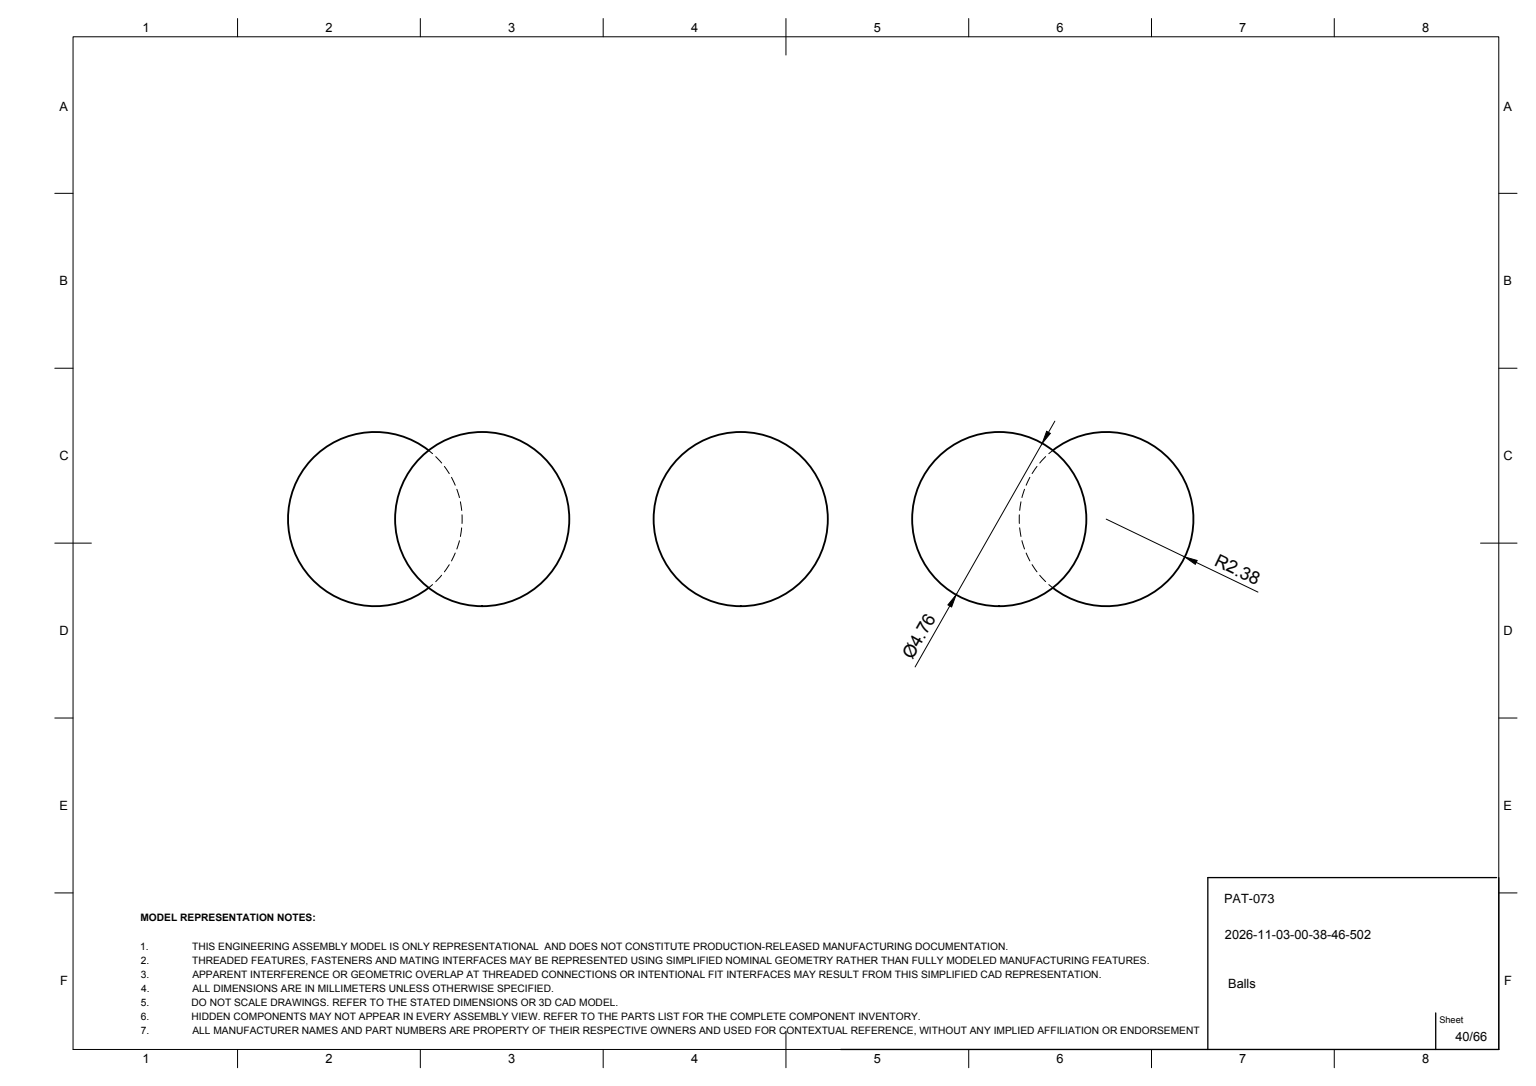
ISO-10303-21;
HEADER;
/* Generated by software containing ST-Developer
 * from STEP Tools, Inc. (www.steptools.com) 
 */

FILE_DESCRIPTION(
/* description */ ('Manual piston pump'),
/* implementation_level */ '2;1');

FILE_NAME(
/* name */ 'Balls.step',
/* time_stamp */ '2026-11-02T16:54:23-08:00',
/* author */ (''),
/* organization */ (''),
/* preprocessor_version */ 'ST-DEVELOPER v20.2',
/* originating_system */ 'Autodesk Translation Framework v15.17.0.0',
/* authorisation */ '');

FILE_SCHEMA (('AUTOMOTIVE_DESIGN { 1 0 10303 214 3 1 1 }'));
ENDSEC;

DATA;
#10=MECHANICAL_DESIGN_GEOMETRIC_PRESENTATION_REPRESENTATION('',(#713,#714,#715,#716,#717,#718,#719,#720),#19043);
#492=SPHERICAL_SURFACE('',#10746,0.23815);
#493=SPHERICAL_SURFACE('',#10748,0.23815);
#494=SPHERICAL_SURFACE('',#10750,0.23815);
#495=SPHERICAL_SURFACE('',#10752,0.23815);
#496=SPHERICAL_SURFACE('',#10754,0.23815);
#497=SPHERICAL_SURFACE('',#10756,0.23815);
#498=SPHERICAL_SURFACE('',#10758,0.23815);
#499=SPHERICAL_SURFACE('',#10760,0.23815);
#587=SHAPE_REPRESENTATION_RELATIONSHIP('SRR','None',#19334,#650);
#650=ADVANCED_BREP_SHAPE_REPRESENTATION('',(#783,#784,#785,#786,#787,#788,
#789,#790),#19001);
#713=STYLED_ITEM('',(#19664),#783);
#714=STYLED_ITEM('',(#19664),#784);
#715=STYLED_ITEM('',(#19664),#785);
#716=STYLED_ITEM('',(#19664),#786);
#717=STYLED_ITEM('',(#19664),#787);
#718=STYLED_ITEM('',(#19664),#788);
#719=STYLED_ITEM('',(#19664),#789);
#720=STYLED_ITEM('',(#19664),#790);
#783=MANIFOLD_SOLID_BREP('Body1',#9499);
#784=MANIFOLD_SOLID_BREP('Body2',#9500);
#785=MANIFOLD_SOLID_BREP('Body3',#9501);
#786=MANIFOLD_SOLID_BREP('Body4',#9502);
#787=MANIFOLD_SOLID_BREP('Body5',#9503);
#788=MANIFOLD_SOLID_BREP('Body6',#9504);
#789=MANIFOLD_SOLID_BREP('Body7',#9505);
#790=MANIFOLD_SOLID_BREP('Body8',#9506);
#1546=FACE_OUTER_BOUND('',#2244,.T.);
#1547=FACE_OUTER_BOUND('',#2245,.T.);
#1548=FACE_OUTER_BOUND('',#2246,.T.);
#1549=FACE_OUTER_BOUND('',#2247,.T.);
#1550=FACE_OUTER_BOUND('',#2248,.T.);
#1551=FACE_OUTER_BOUND('',#2249,.T.);
#1552=FACE_OUTER_BOUND('',#2250,.T.);
#1553=FACE_OUTER_BOUND('',#2251,.T.);
#2244=EDGE_LOOP('',(#7313,#7314));
#2245=EDGE_LOOP('',(#7315,#7316));
#2246=EDGE_LOOP('',(#7317,#7318));
#2247=EDGE_LOOP('',(#7319,#7320));
#2248=EDGE_LOOP('',(#7321,#7322));
#2249=EDGE_LOOP('',(#7323,#7324));
#2250=EDGE_LOOP('',(#7325,#7326));
#2251=EDGE_LOOP('',(#7327,#7328));
#2883=CIRCLE('',#10747,0.23815);
#2884=CIRCLE('',#10749,0.23815);
#2885=CIRCLE('',#10751,0.23815);
#2886=CIRCLE('',#10753,0.23815);
#2887=CIRCLE('',#10755,0.23815);
#2888=CIRCLE('',#10757,0.23815);
#2889=CIRCLE('',#10759,0.23815);
#2890=CIRCLE('',#10761,0.23815);
#4696=VERTEX_POINT('',#15823);
#4697=VERTEX_POINT('',#15824);
#4698=VERTEX_POINT('',#15827);
#4699=VERTEX_POINT('',#15828);
#4700=VERTEX_POINT('',#15831);
#4701=VERTEX_POINT('',#15832);
#4702=VERTEX_POINT('',#15835);
#4703=VERTEX_POINT('',#15836);
#4704=VERTEX_POINT('',#15839);
#4705=VERTEX_POINT('',#15840);
#4706=VERTEX_POINT('',#15843);
#4707=VERTEX_POINT('',#15844);
#4708=VERTEX_POINT('',#15847);
#4709=VERTEX_POINT('',#15848);
#4710=VERTEX_POINT('',#15851);
#4711=VERTEX_POINT('',#15852);
#5643=EDGE_CURVE('',#4696,#4697,#2883,.T.);
#5644=EDGE_CURVE('',#4698,#4699,#2884,.T.);
#5645=EDGE_CURVE('',#4700,#4701,#2885,.T.);
#5646=EDGE_CURVE('',#4702,#4703,#2886,.T.);
#5647=EDGE_CURVE('',#4704,#4705,#2887,.T.);
#5648=EDGE_CURVE('',#4706,#4707,#2888,.T.);
#5649=EDGE_CURVE('',#4708,#4709,#2889,.T.);
#5650=EDGE_CURVE('',#4710,#4711,#2890,.T.);
#7313=ORIENTED_EDGE('',*,*,#5643,.T.);
#7314=ORIENTED_EDGE('',*,*,#5643,.F.);
#7315=ORIENTED_EDGE('',*,*,#5644,.T.);
#7316=ORIENTED_EDGE('',*,*,#5644,.F.);
#7317=ORIENTED_EDGE('',*,*,#5645,.T.);
#7318=ORIENTED_EDGE('',*,*,#5645,.F.);
#7319=ORIENTED_EDGE('',*,*,#5646,.T.);
#7320=ORIENTED_EDGE('',*,*,#5646,.F.);
#7321=ORIENTED_EDGE('',*,*,#5647,.T.);
#7322=ORIENTED_EDGE('',*,*,#5647,.F.);
#7323=ORIENTED_EDGE('',*,*,#5648,.T.);
#7324=ORIENTED_EDGE('',*,*,#5648,.F.);
#7325=ORIENTED_EDGE('',*,*,#5649,.T.);
#7326=ORIENTED_EDGE('',*,*,#5649,.F.);
#7327=ORIENTED_EDGE('',*,*,#5650,.T.);
#7328=ORIENTED_EDGE('',*,*,#5650,.F.);
#9151=ADVANCED_FACE('',(#1546),#492,.T.);
#9152=ADVANCED_FACE('',(#1547),#493,.T.);
#9153=ADVANCED_FACE('',(#1548),#494,.T.);
#9154=ADVANCED_FACE('',(#1549),#495,.T.);
#9155=ADVANCED_FACE('',(#1550),#496,.T.);
#9156=ADVANCED_FACE('',(#1551),#497,.T.);
#9157=ADVANCED_FACE('',(#1552),#498,.T.);
#9158=ADVANCED_FACE('',(#1553),#499,.T.);
#9499=CLOSED_SHELL('',(#9151));
#9500=CLOSED_SHELL('',(#9152));
#9501=CLOSED_SHELL('',(#9153));
#9502=CLOSED_SHELL('',(#9154));
#9503=CLOSED_SHELL('',(#9155));
#9504=CLOSED_SHELL('',(#9156));
#9505=CLOSED_SHELL('',(#9157));
#9506=CLOSED_SHELL('',(#9158));
#10745=AXIS2_PLACEMENT_3D('',#15821,#12784,#12785);
#10746=AXIS2_PLACEMENT_3D('',#15822,#12786,#12787);
#10747=AXIS2_PLACEMENT_3D('',#15825,#12788,#12789);
#10748=AXIS2_PLACEMENT_3D('',#15826,#12790,#12791);
#10749=AXIS2_PLACEMENT_3D('',#15829,#12792,#12793);
#10750=AXIS2_PLACEMENT_3D('',#15830,#12794,#12795);
#10751=AXIS2_PLACEMENT_3D('',#15833,#12796,#12797);
#10752=AXIS2_PLACEMENT_3D('',#15834,#12798,#12799);
#10753=AXIS2_PLACEMENT_3D('',#15837,#12800,#12801);
#10754=AXIS2_PLACEMENT_3D('',#15838,#12802,#12803);
#10755=AXIS2_PLACEMENT_3D('',#15841,#12804,#12805);
#10756=AXIS2_PLACEMENT_3D('',#15842,#12806,#12807);
#10757=AXIS2_PLACEMENT_3D('',#15845,#12808,#12809);
#10758=AXIS2_PLACEMENT_3D('',#15846,#12810,#12811);
#10759=AXIS2_PLACEMENT_3D('',#15849,#12812,#12813);
#10760=AXIS2_PLACEMENT_3D('',#15850,#12814,#12815);
#10761=AXIS2_PLACEMENT_3D('',#15853,#12816,#12817);
#12784=DIRECTION('axis',(0.,0.,1.));
#12785=DIRECTION('refdir',(1.,0.,0.));
#12786=DIRECTION('center_axis',(0.,0.,1.));
#12787=DIRECTION('ref_axis',(1.,0.,0.));
#12788=DIRECTION('center_axis',(1.22464679914735E-16,-1.,0.));
#12789=DIRECTION('ref_axis',(-1.,-1.22464679914735E-16,0.));
#12790=DIRECTION('center_axis',(0.707106781186548,0.,0.707106781186548));
#12791=DIRECTION('ref_axis',(0.707106781186548,0.,-0.707106781186548));
#12792=DIRECTION('center_axis',(8.65956056235494E-17,-1.,-8.65956056235493E-17));
#12793=DIRECTION('ref_axis',(-0.707106781186547,-1.22464679914735E-16,0.707106781186547));
#12794=DIRECTION('center_axis',(1.,0.,0.));
#12795=DIRECTION('ref_axis',(6.12323399573676E-17,0.,-1.));
#12796=DIRECTION('center_axis',(7.49879891330929E-33,-1.,-1.22464679914735E-16));
#12797=DIRECTION('ref_axis',(-6.12323399573676E-17,-1.22464679914735E-16,
1.));
#12798=DIRECTION('center_axis',(0.707106781186548,0.,-0.707106781186548));
#12799=DIRECTION('ref_axis',(-0.707106781186548,0.,-0.707106781186548));
#12800=DIRECTION('center_axis',(-8.65956056235493E-17,-1.,-8.65956056235494E-17));
#12801=DIRECTION('ref_axis',(0.707106781186547,-1.22464679914735E-16,0.707106781186547));
#12802=DIRECTION('center_axis',(0.,0.,-1.));
#12803=DIRECTION('ref_axis',(-1.,0.,-1.22464679914735E-16));
#12804=DIRECTION('center_axis',(-1.22464679914735E-16,-1.,-1.49975978266186E-32));
#12805=DIRECTION('ref_axis',(1.,-1.22464679914735E-16,1.22464679914735E-16));
#12806=DIRECTION('center_axis',(-0.707106781186547,0.,-0.707106781186548));
#12807=DIRECTION('ref_axis',(-0.707106781186548,0.,0.707106781186547));
#12808=DIRECTION('center_axis',(-8.65956056235493E-17,-1.,8.65956056235493E-17));
#12809=DIRECTION('ref_axis',(0.707106781186548,-1.22464679914735E-16,-0.707106781186547));
#12810=DIRECTION('center_axis',(-1.,0.,0.));
#12811=DIRECTION('ref_axis',(-1.83697019872103E-16,0.,1.));
#12812=DIRECTION('center_axis',(-2.24963967399279E-32,-1.,1.22464679914735E-16));
#12813=DIRECTION('ref_axis',(1.83697019872103E-16,-1.22464679914735E-16,
-1.));
#12814=DIRECTION('center_axis',(-0.707106781186548,0.,0.707106781186548));
#12815=DIRECTION('ref_axis',(0.707106781186547,0.,0.707106781186548));
#12816=DIRECTION('center_axis',(8.65956056235493E-17,-1.,8.65956056235493E-17));
#12817=DIRECTION('ref_axis',(-0.707106781186547,-1.22464679914735E-16,-0.707106781186548));
#15821=CARTESIAN_POINT('',(0.,0.,0.));
#15822=CARTESIAN_POINT('Origin',(1.,0.,0.));
#15823=CARTESIAN_POINT('',(1.,-1.78583896120461E-33,0.23815));
#15824=CARTESIAN_POINT('',(1.,-1.78583896120461E-33,-0.23815));
#15825=CARTESIAN_POINT('Origin',(1.,0.,0.));
#15826=CARTESIAN_POINT('Origin',(0.707106781186548,0.,-0.707106781186547));
#15827=CARTESIAN_POINT('',(0.875504261126124,-1.78583896120461E-33,-0.538709301246971));
#15828=CARTESIAN_POINT('',(0.538709301246971,-1.78583896120461E-33,-0.875504261126124));
#15829=CARTESIAN_POINT('Origin',(0.707106781186548,0.,-0.707106781186547));
#15830=CARTESIAN_POINT('Origin',(6.12323399573677E-17,0.,-1.));
#15831=CARTESIAN_POINT('',(0.23815,-1.78583896120461E-33,-1.));
#15832=CARTESIAN_POINT('',(-0.23815,-1.78583896120461E-33,-1.));
#15833=CARTESIAN_POINT('Origin',(6.12323399573677E-17,0.,-1.));
#15834=CARTESIAN_POINT('Origin',(-0.707106781186547,0.,-0.707106781186548));
#15835=CARTESIAN_POINT('',(-0.538709301246971,-1.78583896120461E-33,-0.875504261126124));
#15836=CARTESIAN_POINT('',(-0.875504261126124,-1.78583896120461E-33,-0.538709301246971));
#15837=CARTESIAN_POINT('Origin',(-0.707106781186547,0.,-0.707106781186548));
#15838=CARTESIAN_POINT('Origin',(-1.,0.,-1.22464679914735E-16));
#15839=CARTESIAN_POINT('',(-1.,-1.78583896120461E-33,-0.23815));
#15840=CARTESIAN_POINT('',(-1.,-1.78583896120461E-33,0.23815));
#15841=CARTESIAN_POINT('Origin',(-1.,0.,-1.22464679914735E-16));
#15842=CARTESIAN_POINT('Origin',(-0.707106781186548,0.,0.707106781186547));
#15843=CARTESIAN_POINT('',(-0.875504261126124,-7.94881478324376E-33,0.538709301246971));
#15844=CARTESIAN_POINT('',(-0.538709301246971,4.37713686083455E-33,0.875504261126124));
#15845=CARTESIAN_POINT('Origin',(-0.707106781186548,0.,0.707106781186547));
#15846=CARTESIAN_POINT('Origin',(-1.83697019872103E-16,0.,1.));
#15847=CARTESIAN_POINT('',(-0.23815,-1.78583896120461E-33,1.));
#15848=CARTESIAN_POINT('',(0.23815,-1.78583896120461E-33,1.));
#15849=CARTESIAN_POINT('Origin',(-1.83697019872103E-16,0.,1.));
#15850=CARTESIAN_POINT('Origin',(0.707106781186547,0.,0.707106781186548));
#15851=CARTESIAN_POINT('',(0.538709301246971,-4.86732687222419E-33,0.875504261126124));
#15852=CARTESIAN_POINT('',(0.875504261126124,1.29564894981497E-33,0.538709301246971));
#15853=CARTESIAN_POINT('Origin',(0.707106781186547,0.,0.707106781186548));
#18930=UNCERTAINTY_MEASURE_WITH_UNIT(LENGTH_MEASURE(0.001),#19044,
'DISTANCE_ACCURACY_VALUE',
'Maximum model space distance between geometric entities at asserted c
onnectivities');
#18972=UNCERTAINTY_MEASURE_WITH_UNIT(LENGTH_MEASURE(0.001),#19044,
'DISTANCE_ACCURACY_VALUE',
'Maximum model space distance between geometric entities at asserted c
onnectivities');
#19001=(
GEOMETRIC_REPRESENTATION_CONTEXT(3)
GLOBAL_UNCERTAINTY_ASSIGNED_CONTEXT((#18930))
GLOBAL_UNIT_ASSIGNED_CONTEXT((#19044,#19046,#19047))
REPRESENTATION_CONTEXT('','3D')
);
#19043=(
GEOMETRIC_REPRESENTATION_CONTEXT(3)
GLOBAL_UNCERTAINTY_ASSIGNED_CONTEXT((#18972))
GLOBAL_UNIT_ASSIGNED_CONTEXT((#19044,#19046,#19047))
REPRESENTATION_CONTEXT('','3D')
);
#19044=(
LENGTH_UNIT()
NAMED_UNIT(*)
SI_UNIT(.CENTI.,.METRE.)
);
#19046=(
NAMED_UNIT(*)
PLANE_ANGLE_UNIT()
SI_UNIT($,.RADIAN.)
);
#19047=(
NAMED_UNIT(*)
SI_UNIT($,.STERADIAN.)
SOLID_ANGLE_UNIT()
);
#19076=SHAPE_DEFINITION_REPRESENTATION(#19146,#19334);
#19146=PRODUCT_DEFINITION_SHAPE('',$,#19405);
#19334=SHAPE_REPRESENTATION('',(#10745),#19001);
#19376=PRODUCT_DEFINITION_CONTEXT('part definition',#19588,'design');
#19405=PRODUCT_DEFINITION('2026-11-03-00-38-46-502','Balls',#19475,#19376);
#19475=PRODUCT_DEFINITION_FORMATION('',$,#19618);
#19588=APPLICATION_CONTEXT(
'Core Data for Automotive Mechanical Design Process');
#19589=PRODUCT_CONTEXT('part definition',#19588,'mechanical');
#19618=PRODUCT('2026-11-03-00-38-46-502','Balls','Balls',(#19589));
#19664=PRESENTATION_STYLE_ASSIGNMENT((#19670));
#19670=SURFACE_STYLE_USAGE(.BOTH.,#19676);
#19676=SURFACE_SIDE_STYLE('',(#19682));
#19682=SURFACE_STYLE_FILL_AREA(#19688);
#19688=FILL_AREA_STYLE('CAD Library Painted - Steel gray',(#19694));
#19694=FILL_AREA_STYLE_COLOUR('CAD Library Painted - Steel gray',#19700);
#19700=COLOUR_RGB('CAD Library Painted - Steel gray',0.592156862745098,
0.631372549019608,0.67843137254902);
ENDSEC;
END-ISO-10303-21;
